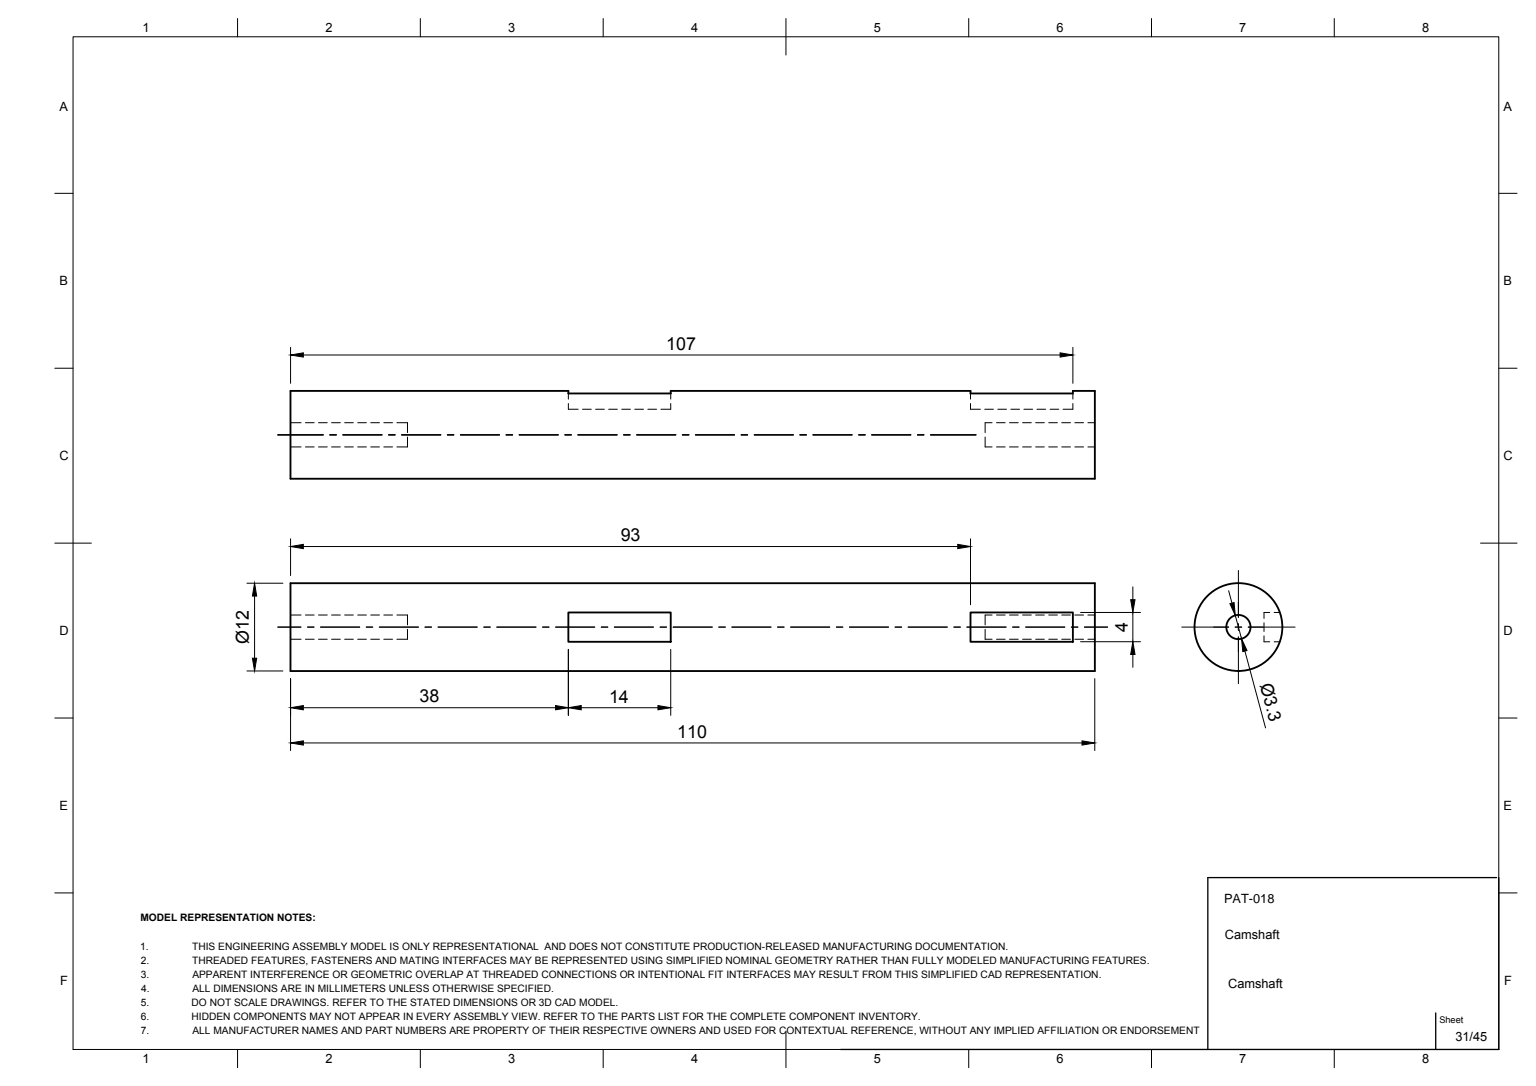
ISO-10303-21;
HEADER;
/* Generated by software containing ST-Developer
 * from STEP Tools, Inc. (www.steptools.com) 
 */

FILE_DESCRIPTION(
/* description */ ('Cam-driven reciprocating slide'),
/* implementation_level */ '2;1');

FILE_NAME(
/* name */ 'Camshaft.step',
/* time_stamp */ '2026-10-28T03:25:20-07:00',
/* author */ (''),
/* organization */ (''),
/* preprocessor_version */ 'ST-DEVELOPER v20.2',
/* originating_system */ 'Autodesk Translation Framework v15.17.0.0',
/* authorisation */ '');

FILE_SCHEMA (('AUTOMOTIVE_DESIGN { 1 0 10303 214 3 1 1 }'));
ENDSEC;

DATA;
#10=MECHANICAL_DESIGN_GEOMETRIC_PRESENTATION_REPRESENTATION('',(#451),#13277);
#370=SHAPE_REPRESENTATION_RELATIONSHIP('SRR','None',#13466,#407);
#407=ADVANCED_BREP_SHAPE_REPRESENTATION('',(#493),#13261);
#451=STYLED_ITEM('',(#13720),#493);
#493=MANIFOLD_SOLID_BREP('Body1',#6429);
#640=FACE_BOUND('',#1685,.T.);
#641=FACE_BOUND('',#1686,.T.);
#642=FACE_BOUND('',#1688,.T.);
#643=FACE_BOUND('',#1690,.T.);
#819=PLANE('',#7389);
#820=PLANE('',#7393);
#821=PLANE('',#7394);
#822=PLANE('',#7395);
#823=PLANE('',#7397);
#824=PLANE('',#7398);
#825=PLANE('',#7399);
#826=PLANE('',#7401);
#827=PLANE('',#7402);
#828=PLANE('',#7404);
#829=PLANE('',#7405);
#830=PLANE('',#7406);
#831=PLANE('',#7411);
#832=PLANE('',#7412);
#1158=FACE_OUTER_BOUND('',#1670,.T.);
#1159=FACE_OUTER_BOUND('',#1671,.T.);
#1160=FACE_OUTER_BOUND('',#1672,.T.);
#1161=FACE_OUTER_BOUND('',#1673,.T.);
#1162=FACE_OUTER_BOUND('',#1674,.T.);
#1163=FACE_OUTER_BOUND('',#1675,.T.);
#1164=FACE_OUTER_BOUND('',#1676,.T.);
#1165=FACE_OUTER_BOUND('',#1677,.T.);
#1166=FACE_OUTER_BOUND('',#1678,.T.);
#1167=FACE_OUTER_BOUND('',#1679,.T.);
#1168=FACE_OUTER_BOUND('',#1680,.T.);
#1169=FACE_OUTER_BOUND('',#1681,.T.);
#1170=FACE_OUTER_BOUND('',#1682,.T.);
#1171=FACE_OUTER_BOUND('',#1683,.T.);
#1172=FACE_OUTER_BOUND('',#1684,.T.);
#1173=FACE_OUTER_BOUND('',#1687,.T.);
#1174=FACE_OUTER_BOUND('',#1689,.T.);
#1670=EDGE_LOOP('',(#5426,#5427,#5428,#5429));
#1671=EDGE_LOOP('',(#5430));
#1672=EDGE_LOOP('',(#5431,#5432,#5433,#5434));
#1673=EDGE_LOOP('',(#5435));
#1674=EDGE_LOOP('',(#5436,#5437,#5438,#5439));
#1675=EDGE_LOOP('',(#5440,#5441,#5442,#5443));
#1676=EDGE_LOOP('',(#5444,#5445,#5446,#5447));
#1677=EDGE_LOOP('',(#5448,#5449,#5450,#5451));
#1678=EDGE_LOOP('',(#5452,#5453,#5454,#5455));
#1679=EDGE_LOOP('',(#5456,#5457,#5458,#5459));
#1680=EDGE_LOOP('',(#5460,#5461,#5462,#5463));
#1681=EDGE_LOOP('',(#5464,#5465,#5466,#5467));
#1682=EDGE_LOOP('',(#5468,#5469,#5470,#5471));
#1683=EDGE_LOOP('',(#5472,#5473,#5474,#5475));
#1684=EDGE_LOOP('',(#5476,#5477,#5478,#5479));
#1685=EDGE_LOOP('',(#5480,#5481,#5482,#5483));
#1686=EDGE_LOOP('',(#5484,#5485,#5486,#5487));
#1687=EDGE_LOOP('',(#5488));
#1688=EDGE_LOOP('',(#5489));
#1689=EDGE_LOOP('',(#5490));
#1690=EDGE_LOOP('',(#5491));
#2121=LINE('',#12606,#2560);
#2122=LINE('',#12613,#2561);
#2123=LINE('',#12619,#2562);
#2124=LINE('',#12621,#2563);
#2125=LINE('',#12623,#2564);
#2126=LINE('',#12624,#2565);
#2127=LINE('',#12629,#2566);
#2128=LINE('',#12630,#2567);
#2129=LINE('',#12633,#2568);
#2130=LINE('',#12635,#2569);
#2131=LINE('',#12636,#2570);
#2132=LINE('',#12638,#2571);
#2133=LINE('',#12644,#2572);
#2134=LINE('',#12646,#2573);
#2135=LINE('',#12648,#2574);
#2136=LINE('',#12649,#2575);
#2137=LINE('',#12654,#2576);
#2138=LINE('',#12655,#2577);
#2139=LINE('',#12658,#2578);
#2140=LINE('',#12660,#2579);
#2141=LINE('',#12661,#2580);
#2142=LINE('',#12663,#2581);
#2143=LINE('',#12670,#2582);
#2560=VECTOR('',#9027,0.165);
#2561=VECTOR('',#9036,0.165);
#2562=VECTOR('',#9043,1.);
#2563=VECTOR('',#9044,1.);
#2564=VECTOR('',#9045,1.);
#2565=VECTOR('',#9046,1.);
#2566=VECTOR('',#9051,1.);
#2567=VECTOR('',#9052,1.);
#2568=VECTOR('',#9055,1.);
#2569=VECTOR('',#9056,1.);
#2570=VECTOR('',#9057,1.);
#2571=VECTOR('',#9060,1.);
#2572=VECTOR('',#9067,1.);
#2573=VECTOR('',#9068,1.);
#2574=VECTOR('',#9069,1.);
#2575=VECTOR('',#9070,1.);
#2576=VECTOR('',#9075,1.);
#2577=VECTOR('',#9076,1.);
#2578=VECTOR('',#9079,1.);
#2579=VECTOR('',#9080,1.);
#2580=VECTOR('',#9081,1.);
#2581=VECTOR('',#9084,1.);
#2582=VECTOR('',#9093,0.6);
#2953=CIRCLE('',#7387,0.165);
#2954=CIRCLE('',#7388,0.165);
#2955=CIRCLE('',#7391,0.165);
#2956=CIRCLE('',#7392,0.165);
#2957=CIRCLE('',#7396,0.6);
#2958=CIRCLE('',#7400,0.6);
#2959=CIRCLE('',#7403,0.6);
#2960=CIRCLE('',#7407,0.6);
#2961=CIRCLE('',#7409,0.6);
#2962=CIRCLE('',#7410,0.6);
#3404=VERTEX_POINT('',#12603);
#3405=VERTEX_POINT('',#12605);
#3406=VERTEX_POINT('',#12610);
#3407=VERTEX_POINT('',#12612);
#3408=VERTEX_POINT('',#12617);
#3409=VERTEX_POINT('',#12618);
#3410=VERTEX_POINT('',#12620);
#3411=VERTEX_POINT('',#12622);
#3412=VERTEX_POINT('',#12626);
#3413=VERTEX_POINT('',#12628);
#3414=VERTEX_POINT('',#12632);
#3415=VERTEX_POINT('',#12634);
#3416=VERTEX_POINT('',#12642);
#3417=VERTEX_POINT('',#12643);
#3418=VERTEX_POINT('',#12645);
#3419=VERTEX_POINT('',#12647);
#3420=VERTEX_POINT('',#12651);
#3421=VERTEX_POINT('',#12653);
#3422=VERTEX_POINT('',#12657);
#3423=VERTEX_POINT('',#12659);
#3424=VERTEX_POINT('',#12667);
#3425=VERTEX_POINT('',#12669);
#4103=EDGE_CURVE('',#3404,#3404,#2953,.T.);
#4104=EDGE_CURVE('',#3404,#3405,#2121,.T.);
#4105=EDGE_CURVE('',#3405,#3405,#2954,.T.);
#4106=EDGE_CURVE('',#3406,#3406,#2955,.T.);
#4107=EDGE_CURVE('',#3406,#3407,#2122,.T.);
#4108=EDGE_CURVE('',#3407,#3407,#2956,.T.);
#4109=EDGE_CURVE('',#3408,#3409,#2123,.T.);
#4110=EDGE_CURVE('',#3408,#3410,#2124,.T.);
#4111=EDGE_CURVE('',#3411,#3410,#2125,.T.);
#4112=EDGE_CURVE('',#3411,#3409,#2126,.T.);
#4113=EDGE_CURVE('',#3409,#3412,#2957,.T.);
#4114=EDGE_CURVE('',#3413,#3411,#2127,.T.);
#4115=EDGE_CURVE('',#3412,#3413,#2128,.T.);
#4116=EDGE_CURVE('',#3412,#3414,#2129,.T.);
#4117=EDGE_CURVE('',#3413,#3415,#2130,.T.);
#4118=EDGE_CURVE('',#3415,#3414,#2131,.T.);
#4119=EDGE_CURVE('',#3410,#3415,#2132,.T.);
#4120=EDGE_CURVE('',#3414,#3408,#2958,.T.);
#4121=EDGE_CURVE('',#3416,#3417,#2133,.T.);
#4122=EDGE_CURVE('',#3416,#3418,#2134,.T.);
#4123=EDGE_CURVE('',#3419,#3418,#2135,.T.);
#4124=EDGE_CURVE('',#3419,#3417,#2136,.T.);
#4125=EDGE_CURVE('',#3417,#3420,#2959,.T.);
#4126=EDGE_CURVE('',#3421,#3419,#2137,.T.);
#4127=EDGE_CURVE('',#3420,#3421,#2138,.T.);
#4128=EDGE_CURVE('',#3420,#3422,#2139,.T.);
#4129=EDGE_CURVE('',#3421,#3423,#2140,.T.);
#4130=EDGE_CURVE('',#3423,#3422,#2141,.T.);
#4131=EDGE_CURVE('',#3418,#3423,#2142,.T.);
#4132=EDGE_CURVE('',#3422,#3416,#2960,.T.);
#4133=EDGE_CURVE('',#3424,#3424,#2961,.T.);
#4134=EDGE_CURVE('',#3424,#3425,#2143,.T.);
#4135=EDGE_CURVE('',#3425,#3425,#2962,.T.);
#5426=ORIENTED_EDGE('',*,*,#4103,.F.);
#5427=ORIENTED_EDGE('',*,*,#4104,.T.);
#5428=ORIENTED_EDGE('',*,*,#4105,.F.);
#5429=ORIENTED_EDGE('',*,*,#4104,.F.);
#5430=ORIENTED_EDGE('',*,*,#4103,.T.);
#5431=ORIENTED_EDGE('',*,*,#4106,.F.);
#5432=ORIENTED_EDGE('',*,*,#4107,.T.);
#5433=ORIENTED_EDGE('',*,*,#4108,.T.);
#5434=ORIENTED_EDGE('',*,*,#4107,.F.);
#5435=ORIENTED_EDGE('',*,*,#4108,.F.);
#5436=ORIENTED_EDGE('',*,*,#4109,.F.);
#5437=ORIENTED_EDGE('',*,*,#4110,.T.);
#5438=ORIENTED_EDGE('',*,*,#4111,.F.);
#5439=ORIENTED_EDGE('',*,*,#4112,.T.);
#5440=ORIENTED_EDGE('',*,*,#4113,.F.);
#5441=ORIENTED_EDGE('',*,*,#4112,.F.);
#5442=ORIENTED_EDGE('',*,*,#4114,.F.);
#5443=ORIENTED_EDGE('',*,*,#4115,.F.);
#5444=ORIENTED_EDGE('',*,*,#4116,.F.);
#5445=ORIENTED_EDGE('',*,*,#4115,.T.);
#5446=ORIENTED_EDGE('',*,*,#4117,.T.);
#5447=ORIENTED_EDGE('',*,*,#4118,.T.);
#5448=ORIENTED_EDGE('',*,*,#4114,.T.);
#5449=ORIENTED_EDGE('',*,*,#4111,.T.);
#5450=ORIENTED_EDGE('',*,*,#4119,.T.);
#5451=ORIENTED_EDGE('',*,*,#4117,.F.);
#5452=ORIENTED_EDGE('',*,*,#4120,.F.);
#5453=ORIENTED_EDGE('',*,*,#4118,.F.);
#5454=ORIENTED_EDGE('',*,*,#4119,.F.);
#5455=ORIENTED_EDGE('',*,*,#4110,.F.);
#5456=ORIENTED_EDGE('',*,*,#4121,.F.);
#5457=ORIENTED_EDGE('',*,*,#4122,.T.);
#5458=ORIENTED_EDGE('',*,*,#4123,.F.);
#5459=ORIENTED_EDGE('',*,*,#4124,.T.);
#5460=ORIENTED_EDGE('',*,*,#4125,.F.);
#5461=ORIENTED_EDGE('',*,*,#4124,.F.);
#5462=ORIENTED_EDGE('',*,*,#4126,.F.);
#5463=ORIENTED_EDGE('',*,*,#4127,.F.);
#5464=ORIENTED_EDGE('',*,*,#4128,.F.);
#5465=ORIENTED_EDGE('',*,*,#4127,.T.);
#5466=ORIENTED_EDGE('',*,*,#4129,.T.);
#5467=ORIENTED_EDGE('',*,*,#4130,.T.);
#5468=ORIENTED_EDGE('',*,*,#4126,.T.);
#5469=ORIENTED_EDGE('',*,*,#4123,.T.);
#5470=ORIENTED_EDGE('',*,*,#4131,.T.);
#5471=ORIENTED_EDGE('',*,*,#4129,.F.);
#5472=ORIENTED_EDGE('',*,*,#4132,.F.);
#5473=ORIENTED_EDGE('',*,*,#4130,.F.);
#5474=ORIENTED_EDGE('',*,*,#4131,.F.);
#5475=ORIENTED_EDGE('',*,*,#4122,.F.);
#5476=ORIENTED_EDGE('',*,*,#4133,.F.);
#5477=ORIENTED_EDGE('',*,*,#4134,.T.);
#5478=ORIENTED_EDGE('',*,*,#4135,.T.);
#5479=ORIENTED_EDGE('',*,*,#4134,.F.);
#5480=ORIENTED_EDGE('',*,*,#4116,.T.);
#5481=ORIENTED_EDGE('',*,*,#4120,.T.);
#5482=ORIENTED_EDGE('',*,*,#4109,.T.);
#5483=ORIENTED_EDGE('',*,*,#4113,.T.);
#5484=ORIENTED_EDGE('',*,*,#4128,.T.);
#5485=ORIENTED_EDGE('',*,*,#4132,.T.);
#5486=ORIENTED_EDGE('',*,*,#4121,.T.);
#5487=ORIENTED_EDGE('',*,*,#4125,.T.);
#5488=ORIENTED_EDGE('',*,*,#4133,.T.);
#5489=ORIENTED_EDGE('',*,*,#4105,.T.);
#5490=ORIENTED_EDGE('',*,*,#4135,.F.);
#5491=ORIENTED_EDGE('',*,*,#4106,.T.);
#5983=CYLINDRICAL_SURFACE('',#7386,0.165);
#5984=CYLINDRICAL_SURFACE('',#7390,0.165);
#5985=CYLINDRICAL_SURFACE('',#7408,0.6);
#6276=ADVANCED_FACE('',(#1158),#5983,.F.);
#6277=ADVANCED_FACE('',(#1159),#819,.T.);
#6278=ADVANCED_FACE('',(#1160),#5984,.F.);
#6279=ADVANCED_FACE('',(#1161),#820,.F.);
#6280=ADVANCED_FACE('',(#1162),#821,.F.);
#6281=ADVANCED_FACE('',(#1163),#822,.T.);
#6282=ADVANCED_FACE('',(#1164),#823,.F.);
#6283=ADVANCED_FACE('',(#1165),#824,.F.);
#6284=ADVANCED_FACE('',(#1166),#825,.F.);
#6285=ADVANCED_FACE('',(#1167),#826,.F.);
#6286=ADVANCED_FACE('',(#1168),#827,.T.);
#6287=ADVANCED_FACE('',(#1169),#828,.F.);
#6288=ADVANCED_FACE('',(#1170),#829,.F.);
#6289=ADVANCED_FACE('',(#1171),#830,.F.);
#6290=ADVANCED_FACE('',(#1172,#640,#641),#5985,.T.);
#6291=ADVANCED_FACE('',(#1173,#642),#831,.T.);
#6292=ADVANCED_FACE('',(#1174,#643),#832,.F.);
#6429=CLOSED_SHELL('',(#6276,#6277,#6278,#6279,#6280,#6281,#6282,#6283,
#6284,#6285,#6286,#6287,#6288,#6289,#6290,#6291,#6292));
#7385=AXIS2_PLACEMENT_3D('',#12601,#9021,#9022);
#7386=AXIS2_PLACEMENT_3D('',#12602,#9023,#9024);
#7387=AXIS2_PLACEMENT_3D('',#12604,#9025,#9026);
#7388=AXIS2_PLACEMENT_3D('',#12607,#9028,#9029);
#7389=AXIS2_PLACEMENT_3D('',#12608,#9030,#9031);
#7390=AXIS2_PLACEMENT_3D('',#12609,#9032,#9033);
#7391=AXIS2_PLACEMENT_3D('',#12611,#9034,#9035);
#7392=AXIS2_PLACEMENT_3D('',#12614,#9037,#9038);
#7393=AXIS2_PLACEMENT_3D('',#12615,#9039,#9040);
#7394=AXIS2_PLACEMENT_3D('',#12616,#9041,#9042);
#7395=AXIS2_PLACEMENT_3D('',#12625,#9047,#9048);
#7396=AXIS2_PLACEMENT_3D('',#12627,#9049,#9050);
#7397=AXIS2_PLACEMENT_3D('',#12631,#9053,#9054);
#7398=AXIS2_PLACEMENT_3D('',#12637,#9058,#9059);
#7399=AXIS2_PLACEMENT_3D('',#12639,#9061,#9062);
#7400=AXIS2_PLACEMENT_3D('',#12640,#9063,#9064);
#7401=AXIS2_PLACEMENT_3D('',#12641,#9065,#9066);
#7402=AXIS2_PLACEMENT_3D('',#12650,#9071,#9072);
#7403=AXIS2_PLACEMENT_3D('',#12652,#9073,#9074);
#7404=AXIS2_PLACEMENT_3D('',#12656,#9077,#9078);
#7405=AXIS2_PLACEMENT_3D('',#12662,#9082,#9083);
#7406=AXIS2_PLACEMENT_3D('',#12664,#9085,#9086);
#7407=AXIS2_PLACEMENT_3D('',#12665,#9087,#9088);
#7408=AXIS2_PLACEMENT_3D('',#12666,#9089,#9090);
#7409=AXIS2_PLACEMENT_3D('',#12668,#9091,#9092);
#7410=AXIS2_PLACEMENT_3D('',#12671,#9094,#9095);
#7411=AXIS2_PLACEMENT_3D('',#12672,#9096,#9097);
#7412=AXIS2_PLACEMENT_3D('',#12673,#9098,#9099);
#9021=DIRECTION('axis',(0.,0.,1.));
#9022=DIRECTION('refdir',(1.,0.,0.));
#9023=DIRECTION('center_axis',(0.,1.,0.));
#9024=DIRECTION('ref_axis',(1.,0.,0.));
#9025=DIRECTION('center_axis',(0.,1.,0.));
#9026=DIRECTION('ref_axis',(1.,0.,0.));
#9027=DIRECTION('',(0.,1.,0.));
#9028=DIRECTION('center_axis',(0.,-1.,0.));
#9029=DIRECTION('ref_axis',(1.,0.,0.));
#9030=DIRECTION('center_axis',(0.,1.,0.));
#9031=DIRECTION('ref_axis',(1.,0.,0.));
#9032=DIRECTION('center_axis',(0.,1.,0.));
#9033=DIRECTION('ref_axis',(1.,0.,0.));
#9034=DIRECTION('center_axis',(0.,1.,0.));
#9035=DIRECTION('ref_axis',(1.,0.,0.));
#9036=DIRECTION('',(0.,1.,0.));
#9037=DIRECTION('center_axis',(0.,1.,0.));
#9038=DIRECTION('ref_axis',(1.,0.,0.));
#9039=DIRECTION('center_axis',(0.,1.,0.));
#9040=DIRECTION('ref_axis',(1.,0.,0.));
#9041=DIRECTION('center_axis',(-1.,0.,0.));
#9042=DIRECTION('ref_axis',(0.,0.,1.));
#9043=DIRECTION('',(0.,-1.,0.));
#9044=DIRECTION('',(0.,0.,1.));
#9045=DIRECTION('',(0.,1.,0.));
#9046=DIRECTION('',(0.,0.,-1.));
#9047=DIRECTION('center_axis',(0.,1.,0.));
#9048=DIRECTION('ref_axis',(1.,0.,0.));
#9049=DIRECTION('center_axis',(0.,-1.,0.));
#9050=DIRECTION('ref_axis',(1.,0.,0.));
#9051=DIRECTION('',(-1.,0.,0.));
#9052=DIRECTION('',(0.,0.,1.));
#9053=DIRECTION('center_axis',(1.,0.,0.));
#9054=DIRECTION('ref_axis',(0.,0.,-1.));
#9055=DIRECTION('',(0.,1.,0.));
#9056=DIRECTION('',(0.,1.,0.));
#9057=DIRECTION('',(0.,0.,-1.));
#9058=DIRECTION('center_axis',(0.,0.,1.));
#9059=DIRECTION('ref_axis',(1.,0.,0.));
#9060=DIRECTION('',(1.,0.,0.));
#9061=DIRECTION('center_axis',(0.,1.,0.));
#9062=DIRECTION('ref_axis',(0.,0.,1.));
#9063=DIRECTION('center_axis',(0.,1.,0.));
#9064=DIRECTION('ref_axis',(1.,0.,0.));
#9065=DIRECTION('center_axis',(-1.,0.,0.));
#9066=DIRECTION('ref_axis',(0.,0.,1.));
#9067=DIRECTION('',(0.,-1.,0.));
#9068=DIRECTION('',(0.,0.,1.));
#9069=DIRECTION('',(0.,1.,0.));
#9070=DIRECTION('',(0.,0.,-1.));
#9071=DIRECTION('center_axis',(0.,1.,0.));
#9072=DIRECTION('ref_axis',(1.,0.,0.));
#9073=DIRECTION('center_axis',(0.,-1.,0.));
#9074=DIRECTION('ref_axis',(1.,0.,0.));
#9075=DIRECTION('',(-1.,0.,0.));
#9076=DIRECTION('',(0.,0.,1.));
#9077=DIRECTION('center_axis',(1.,0.,0.));
#9078=DIRECTION('ref_axis',(0.,0.,-1.));
#9079=DIRECTION('',(0.,1.,0.));
#9080=DIRECTION('',(0.,1.,0.));
#9081=DIRECTION('',(0.,0.,-1.));
#9082=DIRECTION('center_axis',(0.,0.,1.));
#9083=DIRECTION('ref_axis',(1.,0.,0.));
#9084=DIRECTION('',(1.,0.,0.));
#9085=DIRECTION('center_axis',(0.,1.,0.));
#9086=DIRECTION('ref_axis',(0.,0.,1.));
#9087=DIRECTION('center_axis',(0.,1.,0.));
#9088=DIRECTION('ref_axis',(1.,0.,0.));
#9089=DIRECTION('center_axis',(0.,1.,0.));
#9090=DIRECTION('ref_axis',(1.,0.,0.));
#9091=DIRECTION('center_axis',(0.,1.,0.));
#9092=DIRECTION('ref_axis',(1.,0.,0.));
#9093=DIRECTION('',(0.,-1.,0.));
#9094=DIRECTION('center_axis',(0.,1.,0.));
#9095=DIRECTION('ref_axis',(1.,0.,0.));
#9096=DIRECTION('center_axis',(0.,1.,0.));
#9097=DIRECTION('ref_axis',(1.,0.,0.));
#9098=DIRECTION('center_axis',(0.,1.,0.));
#9099=DIRECTION('ref_axis',(1.,0.,0.));
#12601=CARTESIAN_POINT('',(0.,0.,0.));
#12602=CARTESIAN_POINT('Origin',(0.,5.,4.));
#12603=CARTESIAN_POINT('',(-0.165,5.,4.));
#12604=CARTESIAN_POINT('Origin',(0.,5.,4.));
#12605=CARTESIAN_POINT('',(-0.165,6.5,4.));
#12606=CARTESIAN_POINT('',(-0.165,5.,4.));
#12607=CARTESIAN_POINT('Origin',(0.,6.5,4.));
#12608=CARTESIAN_POINT('Origin',(0.,5.,4.));
#12609=CARTESIAN_POINT('Origin',(0.,-4.6,4.));
#12610=CARTESIAN_POINT('',(-0.165,-4.5,4.));
#12611=CARTESIAN_POINT('Origin',(0.,-4.5,4.));
#12612=CARTESIAN_POINT('',(-0.165,-2.9,4.));
#12613=CARTESIAN_POINT('',(-0.165,-4.6,4.));
#12614=CARTESIAN_POINT('Origin',(0.,-2.9,4.));
#12615=CARTESIAN_POINT('Origin',(0.,-2.9,4.));
#12616=CARTESIAN_POINT('Origin',(-0.2,4.8,3.3));
#12617=CARTESIAN_POINT('',(-0.2,6.2,3.43431457505076));
#12618=CARTESIAN_POINT('',(-0.2,4.8,3.43431457505076));
#12619=CARTESIAN_POINT('',(-0.2,-4.5,3.43431457505076));
#12620=CARTESIAN_POINT('',(-0.2,6.2,3.65));
#12621=CARTESIAN_POINT('',(-0.2,6.2,3.65));
#12622=CARTESIAN_POINT('',(-0.2,4.8,3.65));
#12623=CARTESIAN_POINT('',(-0.2,4.8,3.65));
#12624=CARTESIAN_POINT('',(-0.2,4.8,3.65));
#12625=CARTESIAN_POINT('Origin',(0.,4.8,3.475));
#12626=CARTESIAN_POINT('',(0.2,4.8,3.43431457505076));
#12627=CARTESIAN_POINT('Origin',(0.,4.8,4.));
#12628=CARTESIAN_POINT('',(0.2,4.8,3.65));
#12629=CARTESIAN_POINT('',(0.2,4.8,3.65));
#12630=CARTESIAN_POINT('',(0.2,4.8,3.3));
#12631=CARTESIAN_POINT('Origin',(0.2,4.8,3.65));
#12632=CARTESIAN_POINT('',(0.2,6.2,3.43431457505076));
#12633=CARTESIAN_POINT('',(0.2,-4.5,3.43431457505076));
#12634=CARTESIAN_POINT('',(0.2,6.2,3.65));
#12635=CARTESIAN_POINT('',(0.2,4.8,3.65));
#12636=CARTESIAN_POINT('',(0.2,6.2,3.3));
#12637=CARTESIAN_POINT('Origin',(-0.2,4.8,3.65));
#12638=CARTESIAN_POINT('',(0.2,6.2,3.65));
#12639=CARTESIAN_POINT('Origin',(0.,6.2,3.475));
#12640=CARTESIAN_POINT('Origin',(0.,6.2,4.));
#12641=CARTESIAN_POINT('Origin',(-0.2,-0.7,3.3));
#12642=CARTESIAN_POINT('',(-0.2,0.7,3.43431457505076));
#12643=CARTESIAN_POINT('',(-0.2,-0.7,3.43431457505076));
#12644=CARTESIAN_POINT('',(-0.2,-4.5,3.43431457505076));
#12645=CARTESIAN_POINT('',(-0.2,0.7,3.65));
#12646=CARTESIAN_POINT('',(-0.2,0.7,3.65));
#12647=CARTESIAN_POINT('',(-0.2,-0.7,3.65));
#12648=CARTESIAN_POINT('',(-0.2,-0.7,3.65));
#12649=CARTESIAN_POINT('',(-0.2,-0.7,3.65));
#12650=CARTESIAN_POINT('Origin',(0.,-0.7,3.475));
#12651=CARTESIAN_POINT('',(0.2,-0.7,3.43431457505076));
#12652=CARTESIAN_POINT('Origin',(0.,-0.7,4.));
#12653=CARTESIAN_POINT('',(0.2,-0.7,3.65));
#12654=CARTESIAN_POINT('',(0.2,-0.7,3.65));
#12655=CARTESIAN_POINT('',(0.2,-0.7,3.3));
#12656=CARTESIAN_POINT('Origin',(0.2,-0.7,3.65));
#12657=CARTESIAN_POINT('',(0.2,0.7,3.43431457505076));
#12658=CARTESIAN_POINT('',(0.2,-4.5,3.43431457505076));
#12659=CARTESIAN_POINT('',(0.2,0.7,3.65));
#12660=CARTESIAN_POINT('',(0.2,-0.7,3.65));
#12661=CARTESIAN_POINT('',(0.2,0.7,3.3));
#12662=CARTESIAN_POINT('Origin',(-0.2,-0.7,3.65));
#12663=CARTESIAN_POINT('',(0.2,0.7,3.65));
#12664=CARTESIAN_POINT('Origin',(0.,0.7,3.475));
#12665=CARTESIAN_POINT('Origin',(0.,0.7,4.));
#12666=CARTESIAN_POINT('Origin',(0.,-4.5,4.));
#12667=CARTESIAN_POINT('',(-0.6,6.5,4.));
#12668=CARTESIAN_POINT('Origin',(0.,6.5,4.));
#12669=CARTESIAN_POINT('',(-0.6,-4.5,4.));
#12670=CARTESIAN_POINT('',(-0.6,-4.5,4.));
#12671=CARTESIAN_POINT('Origin',(0.,-4.5,4.));
#12672=CARTESIAN_POINT('Origin',(0.,6.5,4.));
#12673=CARTESIAN_POINT('Origin',(0.,-4.5,4.));
#13217=UNCERTAINTY_MEASURE_WITH_UNIT(LENGTH_MEASURE(0.001),#13278,
'DISTANCE_ACCURACY_VALUE',
'Maximum model space distance between geometric entities at asserted c
onnectivities');
#13233=UNCERTAINTY_MEASURE_WITH_UNIT(LENGTH_MEASURE(0.001),#13278,
'DISTANCE_ACCURACY_VALUE',
'Maximum model space distance between geometric entities at asserted c
onnectivities');
#13261=(
GEOMETRIC_REPRESENTATION_CONTEXT(3)
GLOBAL_UNCERTAINTY_ASSIGNED_CONTEXT((#13217))
GLOBAL_UNIT_ASSIGNED_CONTEXT((#13278,#13280,#13281))
REPRESENTATION_CONTEXT('','3D')
);
#13277=(
GEOMETRIC_REPRESENTATION_CONTEXT(3)
GLOBAL_UNCERTAINTY_ASSIGNED_CONTEXT((#13233))
GLOBAL_UNIT_ASSIGNED_CONTEXT((#13278,#13280,#13281))
REPRESENTATION_CONTEXT('','3D')
);
#13278=(
LENGTH_UNIT()
NAMED_UNIT(*)
SI_UNIT(.CENTI.,.METRE.)
);
#13280=(
NAMED_UNIT(*)
PLANE_ANGLE_UNIT()
SI_UNIT($,.RADIAN.)
);
#13281=(
NAMED_UNIT(*)
SI_UNIT($,.STERADIAN.)
SOLID_ANGLE_UNIT()
);
#13309=SHAPE_DEFINITION_REPRESENTATION(#13359,#13466);
#13359=PRODUCT_DEFINITION_SHAPE('',$,#13510);
#13466=SHAPE_REPRESENTATION('',(#7385),#13261);
#13482=PRODUCT_DEFINITION_CONTEXT('part definition',#13613,'design');
#13510=PRODUCT_DEFINITION('Camshaft','Camshaft',#13553,#13482);
#13553=PRODUCT_DEFINITION_FORMATION('',$,#13642);
#13613=APPLICATION_CONTEXT(
'Core Data for Automotive Mechanical Design Process');
#13614=PRODUCT_CONTEXT('part definition',#13613,'mechanical');
#13642=PRODUCT('Camshaft','Camshaft','Camshaft',(#13614));
#13714=COLOUR_RGB('Grey',0.48,0.52,0.57);
#13715=FILL_AREA_STYLE_COLOUR('',#13714);
#13716=FILL_AREA_STYLE('',(#13715));
#13717=SURFACE_STYLE_FILL_AREA(#13716);
#13718=SURFACE_SIDE_STYLE('',(#13717));
#13719=SURFACE_STYLE_USAGE(.BOTH.,#13718);
#13720=PRESENTATION_STYLE_ASSIGNMENT((#13719));
ENDSEC;
END-ISO-10303-21;
